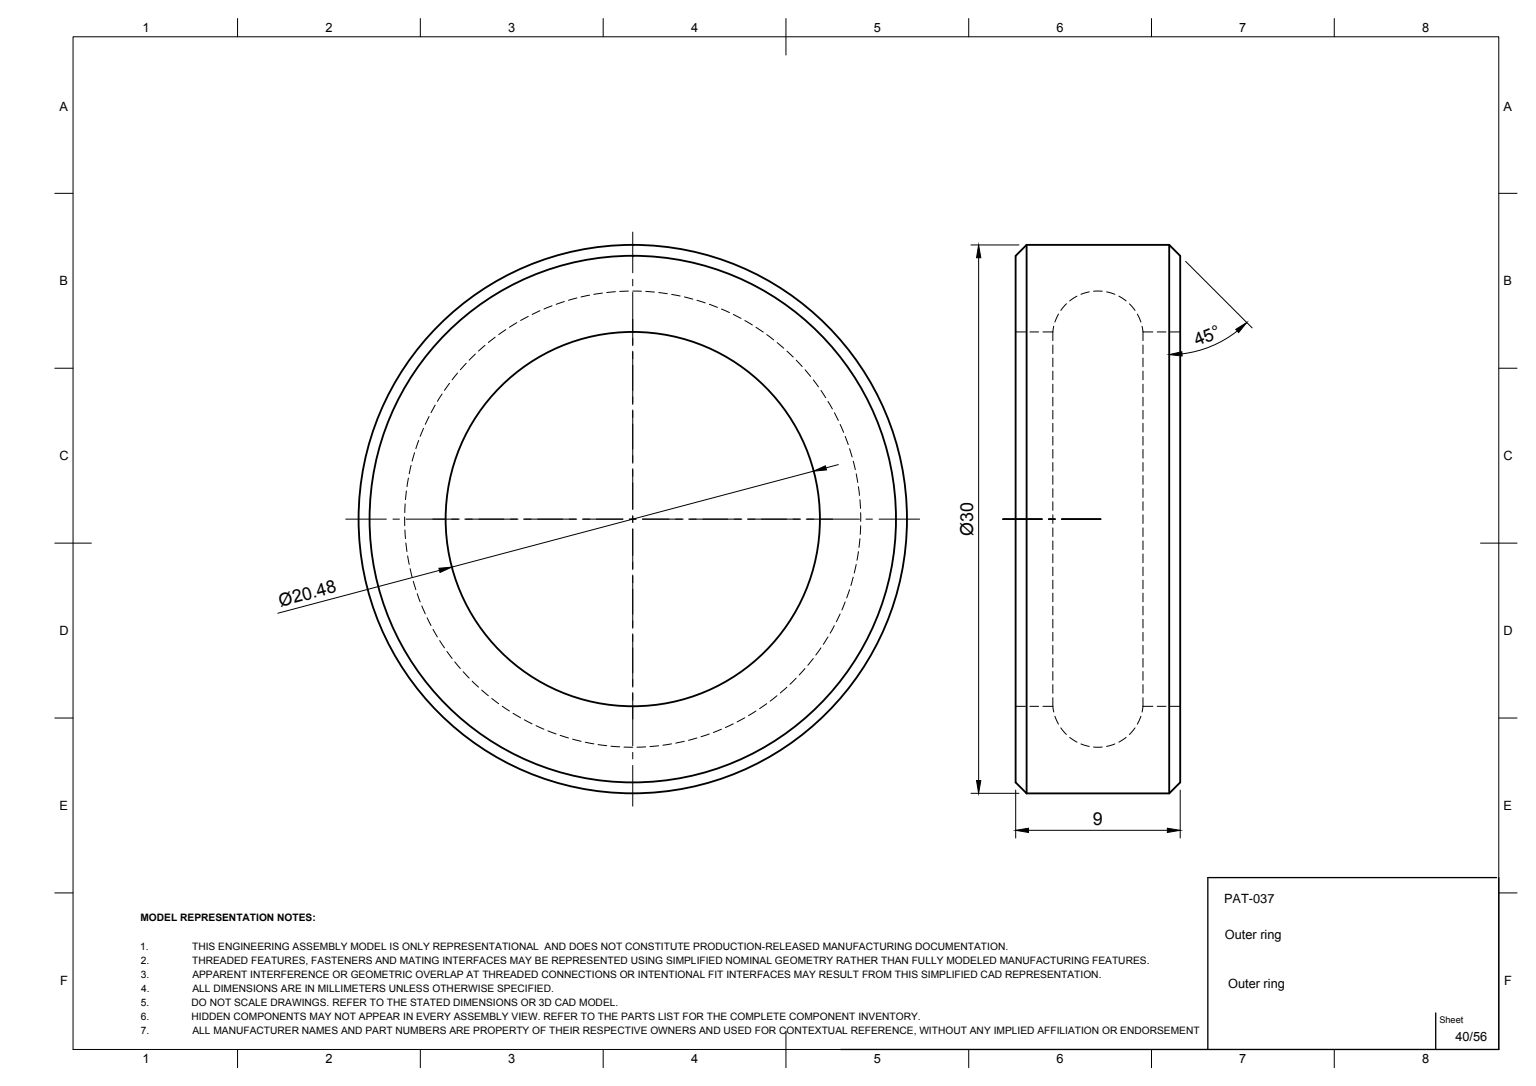
ISO-10303-21;
HEADER;
/* Generated by software containing ST-Developer
 * from STEP Tools, Inc. (www.steptools.com) 
 */

FILE_DESCRIPTION(
/* description */ ('Flywheel Crank-Slider'),
/* implementation_level */ '2;1');

FILE_NAME(
/* name */ 'Outer ring.step',
/* time_stamp */ '2026-10-28T03:23:13-07:00',
/* author */ (''),
/* organization */ (''),
/* preprocessor_version */ 'ST-DEVELOPER v20.2',
/* originating_system */ 'Autodesk Translation Framework v15.17.0.0',
/* authorisation */ '');

FILE_SCHEMA (('AUTOMOTIVE_DESIGN { 1 0 10303 214 3 1 1 }'));
ENDSEC;

DATA;
#10=MECHANICAL_DESIGN_GEOMETRIC_PRESENTATION_REPRESENTATION('',(#707),#17322);
#12=TOROIDAL_SURFACE('',#10415,1.,0.247676);
#554=CONICAL_SURFACE('',#10426,1.47,0.785398163397449);
#555=CONICAL_SURFACE('',#10430,1.47,0.785398163397449);
#602=SHAPE_REPRESENTATION_RELATIONSHIP('SRR','None',#17602,#654);
#654=ADVANCED_BREP_SHAPE_REPRESENTATION('',(#764),#17306);
#707=STYLED_ITEM('',(#17931),#764);
#764=MANIFOLD_SOLID_BREP('Body1',#9089);
#945=FACE_BOUND('',#2408,.T.);
#946=FACE_BOUND('',#2413,.T.);
#1244=PLANE('',#10423);
#1245=PLANE('',#10432);
#1710=FACE_OUTER_BOUND('',#2405,.T.);
#1711=FACE_OUTER_BOUND('',#2406,.T.);
#1712=FACE_OUTER_BOUND('',#2407,.T.);
#1713=FACE_OUTER_BOUND('',#2409,.T.);
#1714=FACE_OUTER_BOUND('',#2410,.T.);
#1715=FACE_OUTER_BOUND('',#2411,.T.);
#1716=FACE_OUTER_BOUND('',#2412,.T.);
#1717=FACE_OUTER_BOUND('',#2414,.T.);
#2405=EDGE_LOOP('',(#7730,#7731,#7732,#7733,#7734,#7735));
#2406=EDGE_LOOP('',(#7736,#7737,#7738,#7739,#7740));
#2407=EDGE_LOOP('',(#7741));
#2408=EDGE_LOOP('',(#7742));
#2409=EDGE_LOOP('',(#7743,#7744,#7745,#7746));
#2410=EDGE_LOOP('',(#7747,#7748,#7749,#7750));
#2411=EDGE_LOOP('',(#7751,#7752,#7753,#7754));
#2412=EDGE_LOOP('',(#7755));
#2413=EDGE_LOOP('',(#7756));
#2414=EDGE_LOOP('',(#7757,#7758,#7759,#7760,#7761));
#3091=LINE('',#16098,#3702);
#3092=LINE('',#16107,#3703);
#3093=LINE('',#16111,#3704);
#3094=LINE('',#16115,#3705);
#3095=LINE('',#16118,#3706);
#3702=VECTOR('',#12781,1.023815);
#3703=VECTOR('',#12792,1.47);
#3704=VECTOR('',#12797,1.5);
#3705=VECTOR('',#12802,1.47);
#3706=VECTOR('',#12807,1.023815);
#4131=CIRCLE('',#10416,1.023815);
#4132=CIRCLE('',#10417,1.023815);
#4133=CIRCLE('',#10418,0.247676);
#4134=CIRCLE('',#10419,1.023815);
#4135=CIRCLE('',#10420,1.023815);
#4136=CIRCLE('',#10422,1.023815);
#4137=CIRCLE('',#10424,1.44);
#4138=CIRCLE('',#10425,1.023815);
#4139=CIRCLE('',#10427,1.5);
#4140=CIRCLE('',#10429,1.5);
#4141=CIRCLE('',#10431,1.44);
#4809=VERTEX_POINT('',#16086);
#4810=VERTEX_POINT('',#16087);
#4811=VERTEX_POINT('',#16090);
#4812=VERTEX_POINT('',#16092);
#4813=VERTEX_POINT('',#16096);
#4814=VERTEX_POINT('',#16100);
#4815=VERTEX_POINT('',#16102);
#4816=VERTEX_POINT('',#16105);
#4817=VERTEX_POINT('',#16109);
#4818=VERTEX_POINT('',#16113);
#5822=EDGE_CURVE('',#4809,#4810,#4131,.T.);
#5823=EDGE_CURVE('',#4810,#4809,#4132,.T.);
#5824=EDGE_CURVE('',#4810,#4811,#4133,.T.);
#5825=EDGE_CURVE('',#4812,#4811,#4134,.T.);
#5826=EDGE_CURVE('',#4811,#4812,#4135,.T.);
#5827=EDGE_CURVE('',#4813,#4813,#4136,.T.);
#5828=EDGE_CURVE('',#4813,#4812,#3091,.T.);
#5829=EDGE_CURVE('',#4814,#4814,#4137,.T.);
#5830=EDGE_CURVE('',#4815,#4815,#4138,.T.);
#5831=EDGE_CURVE('',#4816,#4816,#4139,.T.);
#5832=EDGE_CURVE('',#4816,#4814,#3092,.T.);
#5833=EDGE_CURVE('',#4817,#4817,#4140,.T.);
#5834=EDGE_CURVE('',#4817,#4816,#3093,.T.);
#5835=EDGE_CURVE('',#4818,#4818,#4141,.T.);
#5836=EDGE_CURVE('',#4818,#4817,#3094,.T.);
#5837=EDGE_CURVE('',#4809,#4815,#3095,.T.);
#7730=ORIENTED_EDGE('',*,*,#5822,.F.);
#7731=ORIENTED_EDGE('',*,*,#5823,.F.);
#7732=ORIENTED_EDGE('',*,*,#5824,.T.);
#7733=ORIENTED_EDGE('',*,*,#5825,.F.);
#7734=ORIENTED_EDGE('',*,*,#5826,.F.);
#7735=ORIENTED_EDGE('',*,*,#5824,.F.);
#7736=ORIENTED_EDGE('',*,*,#5827,.T.);
#7737=ORIENTED_EDGE('',*,*,#5828,.T.);
#7738=ORIENTED_EDGE('',*,*,#5825,.T.);
#7739=ORIENTED_EDGE('',*,*,#5826,.T.);
#7740=ORIENTED_EDGE('',*,*,#5828,.F.);
#7741=ORIENTED_EDGE('',*,*,#5829,.F.);
#7742=ORIENTED_EDGE('',*,*,#5830,.T.);
#7743=ORIENTED_EDGE('',*,*,#5831,.F.);
#7744=ORIENTED_EDGE('',*,*,#5832,.T.);
#7745=ORIENTED_EDGE('',*,*,#5829,.T.);
#7746=ORIENTED_EDGE('',*,*,#5832,.F.);
#7747=ORIENTED_EDGE('',*,*,#5833,.F.);
#7748=ORIENTED_EDGE('',*,*,#5834,.T.);
#7749=ORIENTED_EDGE('',*,*,#5831,.T.);
#7750=ORIENTED_EDGE('',*,*,#5834,.F.);
#7751=ORIENTED_EDGE('',*,*,#5835,.F.);
#7752=ORIENTED_EDGE('',*,*,#5836,.T.);
#7753=ORIENTED_EDGE('',*,*,#5833,.T.);
#7754=ORIENTED_EDGE('',*,*,#5836,.F.);
#7755=ORIENTED_EDGE('',*,*,#5835,.T.);
#7756=ORIENTED_EDGE('',*,*,#5827,.F.);
#7757=ORIENTED_EDGE('',*,*,#5822,.T.);
#7758=ORIENTED_EDGE('',*,*,#5823,.T.);
#7759=ORIENTED_EDGE('',*,*,#5837,.T.);
#7760=ORIENTED_EDGE('',*,*,#5830,.F.);
#7761=ORIENTED_EDGE('',*,*,#5837,.F.);
#8464=CYLINDRICAL_SURFACE('',#10421,1.023815);
#8465=CYLINDRICAL_SURFACE('',#10428,1.5);
#8466=CYLINDRICAL_SURFACE('',#10433,1.023815);
#8901=ADVANCED_FACE('',(#1710),#12,.F.);
#8902=ADVANCED_FACE('',(#1711),#8464,.F.);
#8903=ADVANCED_FACE('',(#1712,#945),#1244,.T.);
#8904=ADVANCED_FACE('',(#1713),#554,.T.);
#8905=ADVANCED_FACE('',(#1714),#8465,.T.);
#8906=ADVANCED_FACE('',(#1715),#555,.T.);
#8907=ADVANCED_FACE('',(#1716,#946),#1245,.T.);
#8908=ADVANCED_FACE('',(#1717),#8466,.F.);
#9089=CLOSED_SHELL('',(#8901,#8902,#8903,#8904,#8905,#8906,#8907,#8908));
#10414=AXIS2_PLACEMENT_3D('',#16084,#12763,#12764);
#10415=AXIS2_PLACEMENT_3D('',#16085,#12765,#12766);
#10416=AXIS2_PLACEMENT_3D('',#16088,#12767,#12768);
#10417=AXIS2_PLACEMENT_3D('',#16089,#12769,#12770);
#10418=AXIS2_PLACEMENT_3D('',#16091,#12771,#12772);
#10419=AXIS2_PLACEMENT_3D('',#16093,#12773,#12774);
#10420=AXIS2_PLACEMENT_3D('',#16094,#12775,#12776);
#10421=AXIS2_PLACEMENT_3D('',#16095,#12777,#12778);
#10422=AXIS2_PLACEMENT_3D('',#16097,#12779,#12780);
#10423=AXIS2_PLACEMENT_3D('',#16099,#12782,#12783);
#10424=AXIS2_PLACEMENT_3D('',#16101,#12784,#12785);
#10425=AXIS2_PLACEMENT_3D('',#16103,#12786,#12787);
#10426=AXIS2_PLACEMENT_3D('',#16104,#12788,#12789);
#10427=AXIS2_PLACEMENT_3D('',#16106,#12790,#12791);
#10428=AXIS2_PLACEMENT_3D('',#16108,#12793,#12794);
#10429=AXIS2_PLACEMENT_3D('',#16110,#12795,#12796);
#10430=AXIS2_PLACEMENT_3D('',#16112,#12798,#12799);
#10431=AXIS2_PLACEMENT_3D('',#16114,#12800,#12801);
#10432=AXIS2_PLACEMENT_3D('',#16116,#12803,#12804);
#10433=AXIS2_PLACEMENT_3D('',#16117,#12805,#12806);
#12763=DIRECTION('axis',(0.,0.,1.));
#12764=DIRECTION('refdir',(1.,0.,0.));
#12765=DIRECTION('center_axis',(0.,-1.,0.));
#12766=DIRECTION('ref_axis',(0.,0.,-1.));
#12767=DIRECTION('center_axis',(0.,-1.,0.));
#12768=DIRECTION('ref_axis',(1.,0.,0.));
#12769=DIRECTION('center_axis',(0.,-1.,0.));
#12770=DIRECTION('ref_axis',(1.,0.,0.));
#12771=DIRECTION('center_axis',(1.,0.,1.22464679914735E-16));
#12772=DIRECTION('ref_axis',(-1.22464679914735E-16,0.,1.));
#12773=DIRECTION('center_axis',(0.,1.,0.));
#12774=DIRECTION('ref_axis',(1.,0.,0.));
#12775=DIRECTION('center_axis',(0.,1.,0.));
#12776=DIRECTION('ref_axis',(1.,0.,0.));
#12777=DIRECTION('center_axis',(0.,-1.,0.));
#12778=DIRECTION('ref_axis',(1.,0.,0.));
#12779=DIRECTION('center_axis',(0.,-1.,0.));
#12780=DIRECTION('ref_axis',(1.,0.,0.));
#12781=DIRECTION('',(0.,1.,0.));
#12782=DIRECTION('center_axis',(0.,1.,0.));
#12783=DIRECTION('ref_axis',(0.,0.,1.));
#12784=DIRECTION('center_axis',(0.,-1.,0.));
#12785=DIRECTION('ref_axis',(1.,0.,0.));
#12786=DIRECTION('center_axis',(0.,-1.,0.));
#12787=DIRECTION('ref_axis',(1.,0.,0.));
#12788=DIRECTION('center_axis',(0.,-1.,0.));
#12789=DIRECTION('ref_axis',(1.,0.,0.));
#12790=DIRECTION('center_axis',(0.,-1.,0.));
#12791=DIRECTION('ref_axis',(1.,0.,0.));
#12792=DIRECTION('',(0.707106781186548,0.707106781186547,8.65956056235494E-17));
#12793=DIRECTION('center_axis',(0.,-1.,0.));
#12794=DIRECTION('ref_axis',(1.,0.,0.));
#12795=DIRECTION('center_axis',(0.,-1.,0.));
#12796=DIRECTION('ref_axis',(1.,0.,0.));
#12797=DIRECTION('',(0.,1.,0.));
#12798=DIRECTION('center_axis',(0.,1.,0.));
#12799=DIRECTION('ref_axis',(1.,0.,0.));
#12800=DIRECTION('center_axis',(0.,-1.,0.));
#12801=DIRECTION('ref_axis',(1.,0.,0.));
#12802=DIRECTION('',(-0.707106781186548,0.707106781186547,-8.65956056235494E-17));
#12803=DIRECTION('center_axis',(0.,-1.,0.));
#12804=DIRECTION('ref_axis',(0.,0.,-1.));
#12805=DIRECTION('center_axis',(0.,-1.,0.));
#12806=DIRECTION('ref_axis',(1.,0.,0.));
#12807=DIRECTION('',(0.,1.,0.));
#16084=CARTESIAN_POINT('',(0.,0.,0.));
#16085=CARTESIAN_POINT('Origin',(0.,0.,0.));
#16086=CARTESIAN_POINT('',(-1.023815,0.246528389340863,-1.25381176266905E-16));
#16087=CARTESIAN_POINT('',(-1.25381176266905E-16,0.246528389340863,1.023815));
#16088=CARTESIAN_POINT('Origin',(0.,0.246528389340863,0.));
#16089=CARTESIAN_POINT('Origin',(0.,0.246528389340863,0.));
#16090=CARTESIAN_POINT('',(-1.25381176266905E-16,-0.246528389340863,1.023815));
#16091=CARTESIAN_POINT('Origin',(-1.22464679914735E-16,0.,1.));
#16092=CARTESIAN_POINT('',(-1.023815,-0.246528389340863,1.25381176266905E-16));
#16093=CARTESIAN_POINT('Origin',(0.,-0.246528389340863,0.));
#16094=CARTESIAN_POINT('Origin',(0.,-0.246528389340863,0.));
#16095=CARTESIAN_POINT('Origin',(0.,0.,0.));
#16096=CARTESIAN_POINT('',(-1.023815,-0.45,-1.25381176266905E-16));
#16097=CARTESIAN_POINT('Origin',(0.,-0.45,0.));
#16098=CARTESIAN_POINT('',(-1.023815,0.,-1.25381176266905E-16));
#16099=CARTESIAN_POINT('Origin',(1.44,0.45,0.));
#16100=CARTESIAN_POINT('',(-1.44,0.45,-1.76349139077219E-16));
#16101=CARTESIAN_POINT('Origin',(0.,0.45,0.));
#16102=CARTESIAN_POINT('',(-1.023815,0.45,-1.25381176266905E-16));
#16103=CARTESIAN_POINT('Origin',(0.,0.45,0.));
#16104=CARTESIAN_POINT('Origin',(0.,0.42,0.));
#16105=CARTESIAN_POINT('',(-1.5,0.39,-1.83697019872103E-16));
#16106=CARTESIAN_POINT('Origin',(0.,0.39,0.));
#16107=CARTESIAN_POINT('',(-1.47,0.42,-1.80023079474661E-16));
#16108=CARTESIAN_POINT('Origin',(0.,0.,0.));
#16109=CARTESIAN_POINT('',(-1.5,-0.39,-1.83697019872103E-16));
#16110=CARTESIAN_POINT('Origin',(0.,-0.39,0.));
#16111=CARTESIAN_POINT('',(-1.5,0.,-1.83697019872103E-16));
#16112=CARTESIAN_POINT('Origin',(0.,-0.42,0.));
#16113=CARTESIAN_POINT('',(-1.44,-0.45,-1.76349139077219E-16));
#16114=CARTESIAN_POINT('Origin',(0.,-0.45,0.));
#16115=CARTESIAN_POINT('',(-1.47,-0.42,-1.80023079474661E-16));
#16116=CARTESIAN_POINT('Origin',(1.023815,-0.45,0.));
#16117=CARTESIAN_POINT('Origin',(0.,0.,0.));
#16118=CARTESIAN_POINT('',(-1.023815,0.,-1.25381176266905E-16));
#17245=UNCERTAINTY_MEASURE_WITH_UNIT(LENGTH_MEASURE(0.001),#17323,
'DISTANCE_ACCURACY_VALUE',
'Maximum model space distance between geometric entities at asserted c
onnectivities');
#17261=UNCERTAINTY_MEASURE_WITH_UNIT(LENGTH_MEASURE(0.001),#17323,
'DISTANCE_ACCURACY_VALUE',
'Maximum model space distance between geometric entities at asserted c
onnectivities');
#17306=(
GEOMETRIC_REPRESENTATION_CONTEXT(3)
GLOBAL_UNCERTAINTY_ASSIGNED_CONTEXT((#17245))
GLOBAL_UNIT_ASSIGNED_CONTEXT((#17323,#17325,#17326))
REPRESENTATION_CONTEXT('','3D')
);
#17322=(
GEOMETRIC_REPRESENTATION_CONTEXT(3)
GLOBAL_UNCERTAINTY_ASSIGNED_CONTEXT((#17261))
GLOBAL_UNIT_ASSIGNED_CONTEXT((#17323,#17325,#17326))
REPRESENTATION_CONTEXT('','3D')
);
#17323=(
LENGTH_UNIT()
NAMED_UNIT(*)
SI_UNIT(.CENTI.,.METRE.)
);
#17325=(
NAMED_UNIT(*)
PLANE_ANGLE_UNIT()
SI_UNIT($,.RADIAN.)
);
#17326=(
NAMED_UNIT(*)
SI_UNIT($,.STERADIAN.)
SOLID_ANGLE_UNIT()
);
#17371=SHAPE_DEFINITION_REPRESENTATION(#17433,#17602);
#17433=PRODUCT_DEFINITION_SHAPE('',$,#17663);
#17602=SHAPE_REPRESENTATION('',(#10414),#17306);
#17618=PRODUCT_DEFINITION_CONTEXT('part definition',#17800,'design');
#17663=PRODUCT_DEFINITION('Outer ring','Outer ring',#17723,#17618);
#17723=PRODUCT_DEFINITION_FORMATION('',$,#17846);
#17800=APPLICATION_CONTEXT(
'Core Data for Automotive Mechanical Design Process');
#17801=PRODUCT_CONTEXT('part definition',#17800,'mechanical');
#17846=PRODUCT('Outer ring','Outer ring','Outer ring',(#17801));
#17925=COLOUR_RGB('Grey',0.48,0.52,0.57);
#17926=FILL_AREA_STYLE_COLOUR('',#17925);
#17927=FILL_AREA_STYLE('',(#17926));
#17928=SURFACE_STYLE_FILL_AREA(#17927);
#17929=SURFACE_SIDE_STYLE('',(#17928));
#17930=SURFACE_STYLE_USAGE(.BOTH.,#17929);
#17931=PRESENTATION_STYLE_ASSIGNMENT((#17930));
ENDSEC;
END-ISO-10303-21;
